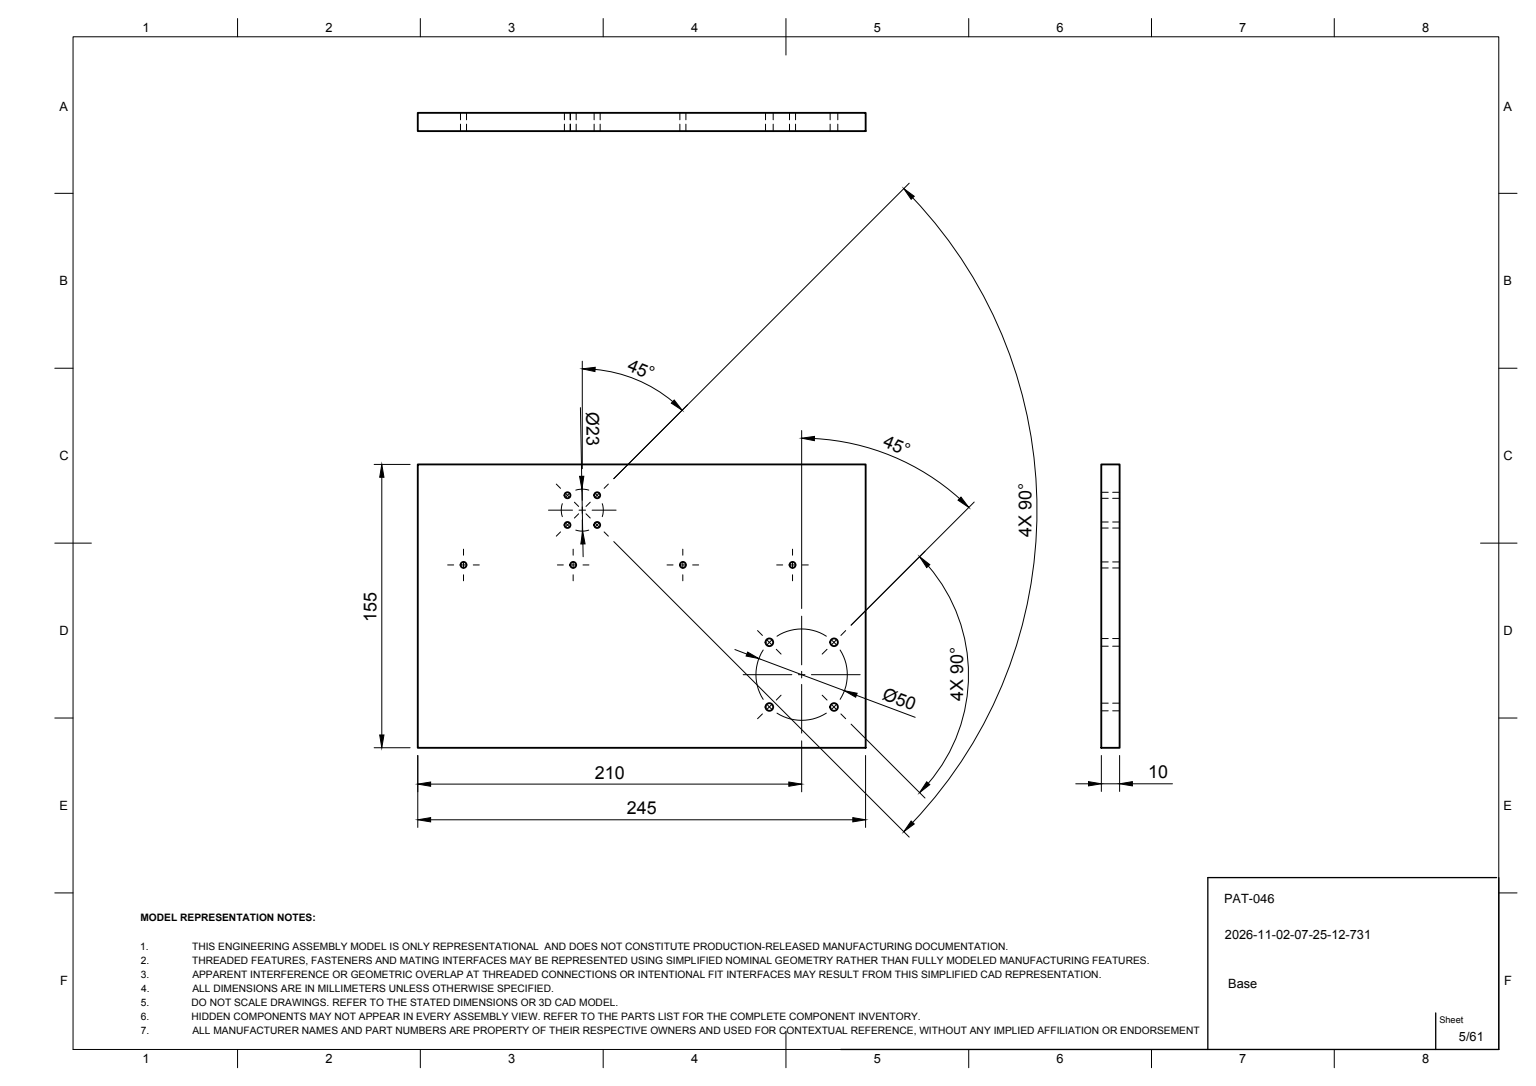
ISO-10303-21;
HEADER;
/* Generated by software containing ST-Developer
 * from STEP Tools, Inc. (www.steptools.com) 
 */

FILE_DESCRIPTION(
/* description */ ('Gear mesh backlash fixture'),
/* implementation_level */ '2;1');

FILE_NAME(
/* name */ 'Base.step',
/* time_stamp */ '2026-10-28T03:26:00-07:00',
/* author */ (''),
/* organization */ (''),
/* preprocessor_version */ 'ST-DEVELOPER v20.2',
/* originating_system */ 'Autodesk Translation Framework v15.17.0.0',
/* authorisation */ '');

FILE_SCHEMA (('AUTOMOTIVE_DESIGN { 1 0 10303 214 3 1 1 }'));
ENDSEC;

DATA;
#10=MECHANICAL_DESIGN_GEOMETRIC_PRESENTATION_REPRESENTATION('',(#1016),#57900);
#916=SHAPE_REPRESENTATION_RELATIONSHIP('SRR','None',#58111,#966);
#966=ADVANCED_BREP_SHAPE_REPRESENTATION('',(#1081),#57844);
#1016=STYLED_ITEM('',(#58444),#1081);
#1081=MANIFOLD_SOLID_BREP('Body1',#13576);
#1143=FACE_BOUND('',#2476,.T.);
#1144=FACE_BOUND('',#2477,.T.);
#1145=FACE_BOUND('',#2478,.T.);
#1146=FACE_BOUND('',#2479,.T.);
#1147=FACE_BOUND('',#2480,.T.);
#1148=FACE_BOUND('',#2481,.T.);
#1149=FACE_BOUND('',#2482,.T.);
#1150=FACE_BOUND('',#2483,.T.);
#1151=FACE_BOUND('',#2484,.T.);
#1152=FACE_BOUND('',#2485,.T.);
#1153=FACE_BOUND('',#2486,.T.);
#1154=FACE_BOUND('',#2487,.T.);
#1155=FACE_BOUND('',#2489,.T.);
#1156=FACE_BOUND('',#2490,.T.);
#1157=FACE_BOUND('',#2491,.T.);
#1158=FACE_BOUND('',#2492,.T.);
#1159=FACE_BOUND('',#2493,.T.);
#1160=FACE_BOUND('',#2494,.T.);
#1161=FACE_BOUND('',#2495,.T.);
#1162=FACE_BOUND('',#2496,.T.);
#1163=FACE_BOUND('',#2497,.T.);
#1164=FACE_BOUND('',#2498,.T.);
#1165=FACE_BOUND('',#2499,.T.);
#1166=FACE_BOUND('',#2500,.T.);
#1330=PLANE('',#14234);
#1331=PLANE('',#14235);
#1332=PLANE('',#14236);
#1333=PLANE('',#14237);
#1334=PLANE('',#14238);
#1335=PLANE('',#14239);
#1694=FACE_OUTER_BOUND('',#2459,.T.);
#1695=FACE_OUTER_BOUND('',#2460,.T.);
#1696=FACE_OUTER_BOUND('',#2461,.T.);
#1697=FACE_OUTER_BOUND('',#2462,.T.);
#1698=FACE_OUTER_BOUND('',#2463,.T.);
#1699=FACE_OUTER_BOUND('',#2464,.T.);
#1700=FACE_OUTER_BOUND('',#2465,.T.);
#1701=FACE_OUTER_BOUND('',#2466,.T.);
#1702=FACE_OUTER_BOUND('',#2467,.T.);
#1703=FACE_OUTER_BOUND('',#2468,.T.);
#1704=FACE_OUTER_BOUND('',#2469,.T.);
#1705=FACE_OUTER_BOUND('',#2470,.T.);
#1706=FACE_OUTER_BOUND('',#2471,.T.);
#1707=FACE_OUTER_BOUND('',#2472,.T.);
#1708=FACE_OUTER_BOUND('',#2473,.T.);
#1709=FACE_OUTER_BOUND('',#2474,.T.);
#1710=FACE_OUTER_BOUND('',#2475,.T.);
#1711=FACE_OUTER_BOUND('',#2488,.T.);
#2459=EDGE_LOOP('',(#8879,#8880,#8881,#8882));
#2460=EDGE_LOOP('',(#8883,#8884,#8885,#8886));
#2461=EDGE_LOOP('',(#8887,#8888,#8889,#8890));
#2462=EDGE_LOOP('',(#8891,#8892,#8893,#8894));
#2463=EDGE_LOOP('',(#8895,#8896,#8897,#8898));
#2464=EDGE_LOOP('',(#8899,#8900,#8901,#8902));
#2465=EDGE_LOOP('',(#8903,#8904,#8905,#8906));
#2466=EDGE_LOOP('',(#8907,#8908,#8909,#8910));
#2467=EDGE_LOOP('',(#8911,#8912,#8913,#8914));
#2468=EDGE_LOOP('',(#8915,#8916,#8917,#8918));
#2469=EDGE_LOOP('',(#8919,#8920,#8921,#8922));
#2470=EDGE_LOOP('',(#8923,#8924,#8925,#8926));
#2471=EDGE_LOOP('',(#8927,#8928,#8929,#8930));
#2472=EDGE_LOOP('',(#8931,#8932,#8933,#8934));
#2473=EDGE_LOOP('',(#8935,#8936,#8937,#8938));
#2474=EDGE_LOOP('',(#8939,#8940,#8941,#8942));
#2475=EDGE_LOOP('',(#8943,#8944,#8945,#8946));
#2476=EDGE_LOOP('',(#8947));
#2477=EDGE_LOOP('',(#8948));
#2478=EDGE_LOOP('',(#8949));
#2479=EDGE_LOOP('',(#8950));
#2480=EDGE_LOOP('',(#8951));
#2481=EDGE_LOOP('',(#8952));
#2482=EDGE_LOOP('',(#8953));
#2483=EDGE_LOOP('',(#8954));
#2484=EDGE_LOOP('',(#8955));
#2485=EDGE_LOOP('',(#8956));
#2486=EDGE_LOOP('',(#8957));
#2487=EDGE_LOOP('',(#8958));
#2488=EDGE_LOOP('',(#8959,#8960,#8961,#8962));
#2489=EDGE_LOOP('',(#8963));
#2490=EDGE_LOOP('',(#8964));
#2491=EDGE_LOOP('',(#8965));
#2492=EDGE_LOOP('',(#8966));
#2493=EDGE_LOOP('',(#8967));
#2494=EDGE_LOOP('',(#8968));
#2495=EDGE_LOOP('',(#8969));
#2496=EDGE_LOOP('',(#8970));
#2497=EDGE_LOOP('',(#8971));
#2498=EDGE_LOOP('',(#8972));
#2499=EDGE_LOOP('',(#8973));
#2500=EDGE_LOOP('',(#8974));
#3411=LINE('',#19240,#4300);
#3412=LINE('',#19246,#4301);
#3413=LINE('',#19252,#4302);
#3414=LINE('',#19258,#4303);
#3415=LINE('',#19264,#4304);
#3416=LINE('',#19270,#4305);
#3417=LINE('',#19276,#4306);
#3418=LINE('',#19282,#4307);
#3419=LINE('',#19288,#4308);
#3420=LINE('',#19294,#4309);
#3421=LINE('',#19300,#4310);
#3422=LINE('',#19306,#4311);
#3423=LINE('',#19311,#4312);
#3424=LINE('',#19313,#4313);
#3425=LINE('',#19315,#4314);
#3426=LINE('',#19316,#4315);
#3427=LINE('',#19319,#4316);
#3428=LINE('',#19321,#4317);
#3429=LINE('',#19322,#4318);
#3430=LINE('',#19325,#4319);
#3431=LINE('',#19327,#4320);
#3432=LINE('',#19328,#4321);
#3433=LINE('',#19330,#4322);
#3434=LINE('',#19331,#4323);
#4300=VECTOR('',#15588,0.164999999999999);
#4301=VECTOR('',#15595,0.164999999999999);
#4302=VECTOR('',#15602,0.164999999999999);
#4303=VECTOR('',#15609,0.164999999999999);
#4304=VECTOR('',#15616,0.21);
#4305=VECTOR('',#15623,0.21);
#4306=VECTOR('',#15630,0.21);
#4307=VECTOR('',#15637,0.21);
#4308=VECTOR('',#15644,0.164999999999999);
#4309=VECTOR('',#15651,0.164999999999999);
#4310=VECTOR('',#15658,0.165);
#4311=VECTOR('',#15665,0.165);
#4312=VECTOR('',#15670,1.);
#4313=VECTOR('',#15671,1.);
#4314=VECTOR('',#15672,1.);
#4315=VECTOR('',#15673,1.);
#4316=VECTOR('',#15676,1.);
#4317=VECTOR('',#15677,1.);
#4318=VECTOR('',#15678,1.);
#4319=VECTOR('',#15681,1.);
#4320=VECTOR('',#15682,1.);
#4321=VECTOR('',#15683,1.);
#4322=VECTOR('',#15686,1.);
#4323=VECTOR('',#15687,1.);
#5189=CIRCLE('',#14199,0.164999999999999);
#5190=CIRCLE('',#14200,0.164999999999999);
#5191=CIRCLE('',#14202,0.164999999999999);
#5192=CIRCLE('',#14203,0.164999999999999);
#5193=CIRCLE('',#14205,0.164999999999999);
#5194=CIRCLE('',#14206,0.164999999999999);
#5195=CIRCLE('',#14208,0.164999999999999);
#5196=CIRCLE('',#14209,0.164999999999999);
#5197=CIRCLE('',#14211,0.21);
#5198=CIRCLE('',#14212,0.21);
#5199=CIRCLE('',#14214,0.21);
#5200=CIRCLE('',#14215,0.21);
#5201=CIRCLE('',#14217,0.21);
#5202=CIRCLE('',#14218,0.21);
#5203=CIRCLE('',#14220,0.21);
#5204=CIRCLE('',#14221,0.21);
#5205=CIRCLE('',#14223,0.164999999999999);
#5206=CIRCLE('',#14224,0.164999999999999);
#5207=CIRCLE('',#14226,0.164999999999999);
#5208=CIRCLE('',#14227,0.164999999999999);
#5209=CIRCLE('',#14229,0.165);
#5210=CIRCLE('',#14230,0.165);
#5211=CIRCLE('',#14232,0.165);
#5212=CIRCLE('',#14233,0.165);
#5781=VERTEX_POINT('',#19237);
#5782=VERTEX_POINT('',#19239);
#5783=VERTEX_POINT('',#19243);
#5784=VERTEX_POINT('',#19245);
#5785=VERTEX_POINT('',#19249);
#5786=VERTEX_POINT('',#19251);
#5787=VERTEX_POINT('',#19255);
#5788=VERTEX_POINT('',#19257);
#5789=VERTEX_POINT('',#19261);
#5790=VERTEX_POINT('',#19263);
#5791=VERTEX_POINT('',#19267);
#5792=VERTEX_POINT('',#19269);
#5793=VERTEX_POINT('',#19273);
#5794=VERTEX_POINT('',#19275);
#5795=VERTEX_POINT('',#19279);
#5796=VERTEX_POINT('',#19281);
#5797=VERTEX_POINT('',#19285);
#5798=VERTEX_POINT('',#19287);
#5799=VERTEX_POINT('',#19291);
#5800=VERTEX_POINT('',#19293);
#5801=VERTEX_POINT('',#19297);
#5802=VERTEX_POINT('',#19299);
#5803=VERTEX_POINT('',#19303);
#5804=VERTEX_POINT('',#19305);
#5805=VERTEX_POINT('',#19309);
#5806=VERTEX_POINT('',#19310);
#5807=VERTEX_POINT('',#19312);
#5808=VERTEX_POINT('',#19314);
#5809=VERTEX_POINT('',#19318);
#5810=VERTEX_POINT('',#19320);
#5811=VERTEX_POINT('',#19324);
#5812=VERTEX_POINT('',#19326);
#7026=EDGE_CURVE('',#5781,#5781,#5189,.T.);
#7027=EDGE_CURVE('',#5781,#5782,#3411,.T.);
#7028=EDGE_CURVE('',#5782,#5782,#5190,.T.);
#7029=EDGE_CURVE('',#5783,#5783,#5191,.T.);
#7030=EDGE_CURVE('',#5783,#5784,#3412,.T.);
#7031=EDGE_CURVE('',#5784,#5784,#5192,.T.);
#7032=EDGE_CURVE('',#5785,#5785,#5193,.T.);
#7033=EDGE_CURVE('',#5785,#5786,#3413,.T.);
#7034=EDGE_CURVE('',#5786,#5786,#5194,.T.);
#7035=EDGE_CURVE('',#5787,#5787,#5195,.T.);
#7036=EDGE_CURVE('',#5787,#5788,#3414,.T.);
#7037=EDGE_CURVE('',#5788,#5788,#5196,.T.);
#7038=EDGE_CURVE('',#5789,#5789,#5197,.T.);
#7039=EDGE_CURVE('',#5789,#5790,#3415,.T.);
#7040=EDGE_CURVE('',#5790,#5790,#5198,.T.);
#7041=EDGE_CURVE('',#5791,#5791,#5199,.T.);
#7042=EDGE_CURVE('',#5791,#5792,#3416,.T.);
#7043=EDGE_CURVE('',#5792,#5792,#5200,.T.);
#7044=EDGE_CURVE('',#5793,#5793,#5201,.T.);
#7045=EDGE_CURVE('',#5793,#5794,#3417,.T.);
#7046=EDGE_CURVE('',#5794,#5794,#5202,.T.);
#7047=EDGE_CURVE('',#5795,#5795,#5203,.T.);
#7048=EDGE_CURVE('',#5795,#5796,#3418,.T.);
#7049=EDGE_CURVE('',#5796,#5796,#5204,.T.);
#7050=EDGE_CURVE('',#5797,#5797,#5205,.T.);
#7051=EDGE_CURVE('',#5797,#5798,#3419,.T.);
#7052=EDGE_CURVE('',#5798,#5798,#5206,.T.);
#7053=EDGE_CURVE('',#5799,#5799,#5207,.T.);
#7054=EDGE_CURVE('',#5799,#5800,#3420,.T.);
#7055=EDGE_CURVE('',#5800,#5800,#5208,.T.);
#7056=EDGE_CURVE('',#5801,#5801,#5209,.T.);
#7057=EDGE_CURVE('',#5801,#5802,#3421,.T.);
#7058=EDGE_CURVE('',#5802,#5802,#5210,.T.);
#7059=EDGE_CURVE('',#5803,#5803,#5211,.T.);
#7060=EDGE_CURVE('',#5803,#5804,#3422,.T.);
#7061=EDGE_CURVE('',#5804,#5804,#5212,.T.);
#7062=EDGE_CURVE('',#5805,#5806,#3423,.T.);
#7063=EDGE_CURVE('',#5806,#5807,#3424,.T.);
#7064=EDGE_CURVE('',#5808,#5807,#3425,.T.);
#7065=EDGE_CURVE('',#5805,#5808,#3426,.T.);
#7066=EDGE_CURVE('',#5809,#5805,#3427,.T.);
#7067=EDGE_CURVE('',#5810,#5808,#3428,.T.);
#7068=EDGE_CURVE('',#5809,#5810,#3429,.T.);
#7069=EDGE_CURVE('',#5811,#5809,#3430,.T.);
#7070=EDGE_CURVE('',#5812,#5810,#3431,.T.);
#7071=EDGE_CURVE('',#5811,#5812,#3432,.T.);
#7072=EDGE_CURVE('',#5806,#5811,#3433,.T.);
#7073=EDGE_CURVE('',#5807,#5812,#3434,.T.);
#8879=ORIENTED_EDGE('',*,*,#7026,.F.);
#8880=ORIENTED_EDGE('',*,*,#7027,.T.);
#8881=ORIENTED_EDGE('',*,*,#7028,.F.);
#8882=ORIENTED_EDGE('',*,*,#7027,.F.);
#8883=ORIENTED_EDGE('',*,*,#7029,.F.);
#8884=ORIENTED_EDGE('',*,*,#7030,.T.);
#8885=ORIENTED_EDGE('',*,*,#7031,.F.);
#8886=ORIENTED_EDGE('',*,*,#7030,.F.);
#8887=ORIENTED_EDGE('',*,*,#7032,.F.);
#8888=ORIENTED_EDGE('',*,*,#7033,.T.);
#8889=ORIENTED_EDGE('',*,*,#7034,.F.);
#8890=ORIENTED_EDGE('',*,*,#7033,.F.);
#8891=ORIENTED_EDGE('',*,*,#7035,.F.);
#8892=ORIENTED_EDGE('',*,*,#7036,.T.);
#8893=ORIENTED_EDGE('',*,*,#7037,.F.);
#8894=ORIENTED_EDGE('',*,*,#7036,.F.);
#8895=ORIENTED_EDGE('',*,*,#7038,.F.);
#8896=ORIENTED_EDGE('',*,*,#7039,.T.);
#8897=ORIENTED_EDGE('',*,*,#7040,.F.);
#8898=ORIENTED_EDGE('',*,*,#7039,.F.);
#8899=ORIENTED_EDGE('',*,*,#7041,.F.);
#8900=ORIENTED_EDGE('',*,*,#7042,.T.);
#8901=ORIENTED_EDGE('',*,*,#7043,.F.);
#8902=ORIENTED_EDGE('',*,*,#7042,.F.);
#8903=ORIENTED_EDGE('',*,*,#7044,.F.);
#8904=ORIENTED_EDGE('',*,*,#7045,.T.);
#8905=ORIENTED_EDGE('',*,*,#7046,.F.);
#8906=ORIENTED_EDGE('',*,*,#7045,.F.);
#8907=ORIENTED_EDGE('',*,*,#7047,.F.);
#8908=ORIENTED_EDGE('',*,*,#7048,.T.);
#8909=ORIENTED_EDGE('',*,*,#7049,.F.);
#8910=ORIENTED_EDGE('',*,*,#7048,.F.);
#8911=ORIENTED_EDGE('',*,*,#7050,.F.);
#8912=ORIENTED_EDGE('',*,*,#7051,.T.);
#8913=ORIENTED_EDGE('',*,*,#7052,.F.);
#8914=ORIENTED_EDGE('',*,*,#7051,.F.);
#8915=ORIENTED_EDGE('',*,*,#7053,.F.);
#8916=ORIENTED_EDGE('',*,*,#7054,.T.);
#8917=ORIENTED_EDGE('',*,*,#7055,.F.);
#8918=ORIENTED_EDGE('',*,*,#7054,.F.);
#8919=ORIENTED_EDGE('',*,*,#7056,.F.);
#8920=ORIENTED_EDGE('',*,*,#7057,.T.);
#8921=ORIENTED_EDGE('',*,*,#7058,.F.);
#8922=ORIENTED_EDGE('',*,*,#7057,.F.);
#8923=ORIENTED_EDGE('',*,*,#7059,.F.);
#8924=ORIENTED_EDGE('',*,*,#7060,.T.);
#8925=ORIENTED_EDGE('',*,*,#7061,.F.);
#8926=ORIENTED_EDGE('',*,*,#7060,.F.);
#8927=ORIENTED_EDGE('',*,*,#7062,.T.);
#8928=ORIENTED_EDGE('',*,*,#7063,.T.);
#8929=ORIENTED_EDGE('',*,*,#7064,.F.);
#8930=ORIENTED_EDGE('',*,*,#7065,.F.);
#8931=ORIENTED_EDGE('',*,*,#7066,.T.);
#8932=ORIENTED_EDGE('',*,*,#7065,.T.);
#8933=ORIENTED_EDGE('',*,*,#7067,.F.);
#8934=ORIENTED_EDGE('',*,*,#7068,.F.);
#8935=ORIENTED_EDGE('',*,*,#7069,.T.);
#8936=ORIENTED_EDGE('',*,*,#7068,.T.);
#8937=ORIENTED_EDGE('',*,*,#7070,.F.);
#8938=ORIENTED_EDGE('',*,*,#7071,.F.);
#8939=ORIENTED_EDGE('',*,*,#7072,.T.);
#8940=ORIENTED_EDGE('',*,*,#7071,.T.);
#8941=ORIENTED_EDGE('',*,*,#7073,.F.);
#8942=ORIENTED_EDGE('',*,*,#7063,.F.);
#8943=ORIENTED_EDGE('',*,*,#7073,.T.);
#8944=ORIENTED_EDGE('',*,*,#7070,.T.);
#8945=ORIENTED_EDGE('',*,*,#7067,.T.);
#8946=ORIENTED_EDGE('',*,*,#7064,.T.);
#8947=ORIENTED_EDGE('',*,*,#7040,.T.);
#8948=ORIENTED_EDGE('',*,*,#7043,.T.);
#8949=ORIENTED_EDGE('',*,*,#7046,.T.);
#8950=ORIENTED_EDGE('',*,*,#7049,.T.);
#8951=ORIENTED_EDGE('',*,*,#7052,.T.);
#8952=ORIENTED_EDGE('',*,*,#7055,.T.);
#8953=ORIENTED_EDGE('',*,*,#7058,.T.);
#8954=ORIENTED_EDGE('',*,*,#7061,.T.);
#8955=ORIENTED_EDGE('',*,*,#7037,.T.);
#8956=ORIENTED_EDGE('',*,*,#7034,.T.);
#8957=ORIENTED_EDGE('',*,*,#7031,.T.);
#8958=ORIENTED_EDGE('',*,*,#7028,.T.);
#8959=ORIENTED_EDGE('',*,*,#7072,.F.);
#8960=ORIENTED_EDGE('',*,*,#7062,.F.);
#8961=ORIENTED_EDGE('',*,*,#7066,.F.);
#8962=ORIENTED_EDGE('',*,*,#7069,.F.);
#8963=ORIENTED_EDGE('',*,*,#7038,.T.);
#8964=ORIENTED_EDGE('',*,*,#7041,.T.);
#8965=ORIENTED_EDGE('',*,*,#7044,.T.);
#8966=ORIENTED_EDGE('',*,*,#7047,.T.);
#8967=ORIENTED_EDGE('',*,*,#7050,.T.);
#8968=ORIENTED_EDGE('',*,*,#7053,.T.);
#8969=ORIENTED_EDGE('',*,*,#7056,.T.);
#8970=ORIENTED_EDGE('',*,*,#7059,.T.);
#8971=ORIENTED_EDGE('',*,*,#7035,.T.);
#8972=ORIENTED_EDGE('',*,*,#7032,.T.);
#8973=ORIENTED_EDGE('',*,*,#7029,.T.);
#8974=ORIENTED_EDGE('',*,*,#7026,.T.);
#12585=CYLINDRICAL_SURFACE('',#14198,0.164999999999999);
#12586=CYLINDRICAL_SURFACE('',#14201,0.164999999999999);
#12587=CYLINDRICAL_SURFACE('',#14204,0.164999999999999);
#12588=CYLINDRICAL_SURFACE('',#14207,0.164999999999999);
#12589=CYLINDRICAL_SURFACE('',#14210,0.21);
#12590=CYLINDRICAL_SURFACE('',#14213,0.21);
#12591=CYLINDRICAL_SURFACE('',#14216,0.21);
#12592=CYLINDRICAL_SURFACE('',#14219,0.21);
#12593=CYLINDRICAL_SURFACE('',#14222,0.164999999999999);
#12594=CYLINDRICAL_SURFACE('',#14225,0.164999999999999);
#12595=CYLINDRICAL_SURFACE('',#14228,0.165);
#12596=CYLINDRICAL_SURFACE('',#14231,0.165);
#12811=ADVANCED_FACE('',(#1694),#12585,.F.);
#12812=ADVANCED_FACE('',(#1695),#12586,.F.);
#12813=ADVANCED_FACE('',(#1696),#12587,.F.);
#12814=ADVANCED_FACE('',(#1697),#12588,.F.);
#12815=ADVANCED_FACE('',(#1698),#12589,.F.);
#12816=ADVANCED_FACE('',(#1699),#12590,.F.);
#12817=ADVANCED_FACE('',(#1700),#12591,.F.);
#12818=ADVANCED_FACE('',(#1701),#12592,.F.);
#12819=ADVANCED_FACE('',(#1702),#12593,.F.);
#12820=ADVANCED_FACE('',(#1703),#12594,.F.);
#12821=ADVANCED_FACE('',(#1704),#12595,.F.);
#12822=ADVANCED_FACE('',(#1705),#12596,.F.);
#12823=ADVANCED_FACE('',(#1706),#1330,.T.);
#12824=ADVANCED_FACE('',(#1707),#1331,.T.);
#12825=ADVANCED_FACE('',(#1708),#1332,.T.);
#12826=ADVANCED_FACE('',(#1709),#1333,.T.);
#12827=ADVANCED_FACE('',(#1710,#1143,#1144,#1145,#1146,#1147,#1148,#1149,
#1150,#1151,#1152,#1153,#1154),#1334,.T.);
#12828=ADVANCED_FACE('',(#1711,#1155,#1156,#1157,#1158,#1159,#1160,#1161,
#1162,#1163,#1164,#1165,#1166),#1335,.F.);
#13576=CLOSED_SHELL('',(#12811,#12812,#12813,#12814,#12815,#12816,#12817,
#12818,#12819,#12820,#12821,#12822,#12823,#12824,#12825,#12826,#12827,#12828));
#14197=AXIS2_PLACEMENT_3D('',#19235,#15582,#15583);
#14198=AXIS2_PLACEMENT_3D('',#19236,#15584,#15585);
#14199=AXIS2_PLACEMENT_3D('',#19238,#15586,#15587);
#14200=AXIS2_PLACEMENT_3D('',#19241,#15589,#15590);
#14201=AXIS2_PLACEMENT_3D('',#19242,#15591,#15592);
#14202=AXIS2_PLACEMENT_3D('',#19244,#15593,#15594);
#14203=AXIS2_PLACEMENT_3D('',#19247,#15596,#15597);
#14204=AXIS2_PLACEMENT_3D('',#19248,#15598,#15599);
#14205=AXIS2_PLACEMENT_3D('',#19250,#15600,#15601);
#14206=AXIS2_PLACEMENT_3D('',#19253,#15603,#15604);
#14207=AXIS2_PLACEMENT_3D('',#19254,#15605,#15606);
#14208=AXIS2_PLACEMENT_3D('',#19256,#15607,#15608);
#14209=AXIS2_PLACEMENT_3D('',#19259,#15610,#15611);
#14210=AXIS2_PLACEMENT_3D('',#19260,#15612,#15613);
#14211=AXIS2_PLACEMENT_3D('',#19262,#15614,#15615);
#14212=AXIS2_PLACEMENT_3D('',#19265,#15617,#15618);
#14213=AXIS2_PLACEMENT_3D('',#19266,#15619,#15620);
#14214=AXIS2_PLACEMENT_3D('',#19268,#15621,#15622);
#14215=AXIS2_PLACEMENT_3D('',#19271,#15624,#15625);
#14216=AXIS2_PLACEMENT_3D('',#19272,#15626,#15627);
#14217=AXIS2_PLACEMENT_3D('',#19274,#15628,#15629);
#14218=AXIS2_PLACEMENT_3D('',#19277,#15631,#15632);
#14219=AXIS2_PLACEMENT_3D('',#19278,#15633,#15634);
#14220=AXIS2_PLACEMENT_3D('',#19280,#15635,#15636);
#14221=AXIS2_PLACEMENT_3D('',#19283,#15638,#15639);
#14222=AXIS2_PLACEMENT_3D('',#19284,#15640,#15641);
#14223=AXIS2_PLACEMENT_3D('',#19286,#15642,#15643);
#14224=AXIS2_PLACEMENT_3D('',#19289,#15645,#15646);
#14225=AXIS2_PLACEMENT_3D('',#19290,#15647,#15648);
#14226=AXIS2_PLACEMENT_3D('',#19292,#15649,#15650);
#14227=AXIS2_PLACEMENT_3D('',#19295,#15652,#15653);
#14228=AXIS2_PLACEMENT_3D('',#19296,#15654,#15655);
#14229=AXIS2_PLACEMENT_3D('',#19298,#15656,#15657);
#14230=AXIS2_PLACEMENT_3D('',#19301,#15659,#15660);
#14231=AXIS2_PLACEMENT_3D('',#19302,#15661,#15662);
#14232=AXIS2_PLACEMENT_3D('',#19304,#15663,#15664);
#14233=AXIS2_PLACEMENT_3D('',#19307,#15666,#15667);
#14234=AXIS2_PLACEMENT_3D('',#19308,#15668,#15669);
#14235=AXIS2_PLACEMENT_3D('',#19317,#15674,#15675);
#14236=AXIS2_PLACEMENT_3D('',#19323,#15679,#15680);
#14237=AXIS2_PLACEMENT_3D('',#19329,#15684,#15685);
#14238=AXIS2_PLACEMENT_3D('',#19332,#15688,#15689);
#14239=AXIS2_PLACEMENT_3D('',#19333,#15690,#15691);
#15582=DIRECTION('axis',(0.,0.,1.));
#15583=DIRECTION('refdir',(1.,0.,0.));
#15584=DIRECTION('center_axis',(0.,0.,1.));
#15585=DIRECTION('ref_axis',(1.,0.,0.));
#15586=DIRECTION('center_axis',(0.,0.,1.));
#15587=DIRECTION('ref_axis',(1.,0.,0.));
#15588=DIRECTION('',(0.,0.,1.));
#15589=DIRECTION('center_axis',(0.,0.,-1.));
#15590=DIRECTION('ref_axis',(1.,0.,0.));
#15591=DIRECTION('center_axis',(0.,0.,1.));
#15592=DIRECTION('ref_axis',(1.,0.,0.));
#15593=DIRECTION('center_axis',(0.,0.,1.));
#15594=DIRECTION('ref_axis',(1.,0.,0.));
#15595=DIRECTION('',(0.,0.,1.));
#15596=DIRECTION('center_axis',(0.,0.,-1.));
#15597=DIRECTION('ref_axis',(1.,0.,0.));
#15598=DIRECTION('center_axis',(0.,0.,1.));
#15599=DIRECTION('ref_axis',(1.,0.,0.));
#15600=DIRECTION('center_axis',(0.,0.,1.));
#15601=DIRECTION('ref_axis',(1.,0.,0.));
#15602=DIRECTION('',(0.,0.,1.));
#15603=DIRECTION('center_axis',(0.,0.,-1.));
#15604=DIRECTION('ref_axis',(1.,0.,0.));
#15605=DIRECTION('center_axis',(0.,0.,1.));
#15606=DIRECTION('ref_axis',(1.,0.,0.));
#15607=DIRECTION('center_axis',(0.,0.,1.));
#15608=DIRECTION('ref_axis',(1.,0.,0.));
#15609=DIRECTION('',(0.,0.,1.));
#15610=DIRECTION('center_axis',(0.,0.,-1.));
#15611=DIRECTION('ref_axis',(1.,0.,0.));
#15612=DIRECTION('center_axis',(0.,0.,1.));
#15613=DIRECTION('ref_axis',(1.,0.,0.));
#15614=DIRECTION('center_axis',(0.,0.,1.));
#15615=DIRECTION('ref_axis',(1.,0.,0.));
#15616=DIRECTION('',(0.,0.,1.));
#15617=DIRECTION('center_axis',(0.,0.,-1.));
#15618=DIRECTION('ref_axis',(1.,0.,0.));
#15619=DIRECTION('center_axis',(0.,0.,1.));
#15620=DIRECTION('ref_axis',(1.,0.,0.));
#15621=DIRECTION('center_axis',(0.,0.,1.));
#15622=DIRECTION('ref_axis',(1.,0.,0.));
#15623=DIRECTION('',(0.,0.,1.));
#15624=DIRECTION('center_axis',(0.,0.,-1.));
#15625=DIRECTION('ref_axis',(1.,0.,0.));
#15626=DIRECTION('center_axis',(0.,0.,1.));
#15627=DIRECTION('ref_axis',(1.,0.,0.));
#15628=DIRECTION('center_axis',(0.,0.,1.));
#15629=DIRECTION('ref_axis',(1.,0.,0.));
#15630=DIRECTION('',(0.,0.,1.));
#15631=DIRECTION('center_axis',(0.,0.,-1.));
#15632=DIRECTION('ref_axis',(1.,0.,0.));
#15633=DIRECTION('center_axis',(0.,0.,1.));
#15634=DIRECTION('ref_axis',(1.,0.,0.));
#15635=DIRECTION('center_axis',(0.,0.,1.));
#15636=DIRECTION('ref_axis',(1.,0.,0.));
#15637=DIRECTION('',(0.,0.,1.));
#15638=DIRECTION('center_axis',(0.,0.,-1.));
#15639=DIRECTION('ref_axis',(1.,0.,0.));
#15640=DIRECTION('center_axis',(0.,0.,1.));
#15641=DIRECTION('ref_axis',(1.,0.,0.));
#15642=DIRECTION('center_axis',(0.,0.,1.));
#15643=DIRECTION('ref_axis',(1.,0.,0.));
#15644=DIRECTION('',(0.,0.,1.));
#15645=DIRECTION('center_axis',(0.,0.,-1.));
#15646=DIRECTION('ref_axis',(1.,0.,0.));
#15647=DIRECTION('center_axis',(0.,0.,1.));
#15648=DIRECTION('ref_axis',(1.,0.,0.));
#15649=DIRECTION('center_axis',(0.,0.,1.));
#15650=DIRECTION('ref_axis',(1.,0.,0.));
#15651=DIRECTION('',(0.,0.,1.));
#15652=DIRECTION('center_axis',(0.,0.,-1.));
#15653=DIRECTION('ref_axis',(1.,0.,0.));
#15654=DIRECTION('center_axis',(0.,0.,1.));
#15655=DIRECTION('ref_axis',(1.,0.,0.));
#15656=DIRECTION('center_axis',(0.,0.,1.));
#15657=DIRECTION('ref_axis',(1.,0.,0.));
#15658=DIRECTION('',(0.,0.,1.));
#15659=DIRECTION('center_axis',(0.,0.,-1.));
#15660=DIRECTION('ref_axis',(1.,0.,0.));
#15661=DIRECTION('center_axis',(0.,0.,1.));
#15662=DIRECTION('ref_axis',(1.,0.,0.));
#15663=DIRECTION('center_axis',(0.,0.,1.));
#15664=DIRECTION('ref_axis',(1.,0.,0.));
#15665=DIRECTION('',(0.,0.,1.));
#15666=DIRECTION('center_axis',(0.,0.,-1.));
#15667=DIRECTION('ref_axis',(1.,0.,0.));
#15668=DIRECTION('center_axis',(0.,1.,0.));
#15669=DIRECTION('ref_axis',(-1.,0.,0.));
#15670=DIRECTION('',(-1.,0.,0.));
#15671=DIRECTION('',(0.,0.,1.));
#15672=DIRECTION('',(-1.,0.,0.));
#15673=DIRECTION('',(0.,0.,1.));
#15674=DIRECTION('center_axis',(1.,0.,0.));
#15675=DIRECTION('ref_axis',(0.,1.,0.));
#15676=DIRECTION('',(0.,1.,0.));
#15677=DIRECTION('',(0.,1.,0.));
#15678=DIRECTION('',(0.,0.,1.));
#15679=DIRECTION('center_axis',(0.,-1.,0.));
#15680=DIRECTION('ref_axis',(1.,0.,0.));
#15681=DIRECTION('',(1.,0.,0.));
#15682=DIRECTION('',(1.,0.,0.));
#15683=DIRECTION('',(0.,0.,1.));
#15684=DIRECTION('center_axis',(-1.,0.,0.));
#15685=DIRECTION('ref_axis',(0.,-1.,0.));
#15686=DIRECTION('',(0.,-1.,0.));
#15687=DIRECTION('',(0.,-1.,0.));
#15688=DIRECTION('center_axis',(0.,0.,1.));
#15689=DIRECTION('ref_axis',(1.,0.,0.));
#15690=DIRECTION('center_axis',(0.,0.,1.));
#15691=DIRECTION('ref_axis',(1.,0.,0.));
#19235=CARTESIAN_POINT('',(0.,0.,0.));
#19236=CARTESIAN_POINT('Origin',(11.1868272016355,8.18682720163547,-1.1));
#19237=CARTESIAN_POINT('',(11.0218272016355,8.18682720163547,-1.));
#19238=CARTESIAN_POINT('Origin',(11.1868272016355,8.18682720163547,-1.));
#19239=CARTESIAN_POINT('',(11.0218272016355,8.18682720163547,0.));
#19240=CARTESIAN_POINT('',(11.0218272016355,8.18682720163547,-1.1));
#19241=CARTESIAN_POINT('Origin',(11.1868272016355,8.18682720163547,0.));
#19242=CARTESIAN_POINT('Origin',(11.1868272016355,9.81317279836453,-1.1));
#19243=CARTESIAN_POINT('',(11.0218272016355,9.81317279836453,-1.));
#19244=CARTESIAN_POINT('Origin',(11.1868272016355,9.81317279836453,-1.));
#19245=CARTESIAN_POINT('',(11.0218272016355,9.81317279836453,0.));
#19246=CARTESIAN_POINT('',(11.0218272016355,9.81317279836453,-1.1));
#19247=CARTESIAN_POINT('Origin',(11.1868272016355,9.81317279836453,0.));
#19248=CARTESIAN_POINT('Origin',(12.8131727983645,9.81317279836453,-1.1));
#19249=CARTESIAN_POINT('',(12.6481727983645,9.81317279836453,-1.));
#19250=CARTESIAN_POINT('Origin',(12.8131727983645,9.81317279836453,-1.));
#19251=CARTESIAN_POINT('',(12.6481727983645,9.81317279836453,0.));
#19252=CARTESIAN_POINT('',(12.6481727983645,9.81317279836453,-1.1));
#19253=CARTESIAN_POINT('Origin',(12.8131727983645,9.81317279836453,0.));
#19254=CARTESIAN_POINT('Origin',(12.8131727983645,8.18682720163547,-1.1));
#19255=CARTESIAN_POINT('',(12.6481727983645,8.18682720163547,-1.));
#19256=CARTESIAN_POINT('Origin',(12.8131727983645,8.18682720163547,-1.));
#19257=CARTESIAN_POINT('',(12.6481727983645,8.18682720163547,0.));
#19258=CARTESIAN_POINT('',(12.6481727983645,8.18682720163547,-1.1));
#19259=CARTESIAN_POINT('Origin',(12.8131727983645,8.18682720163547,0.));
#19260=CARTESIAN_POINT('Origin',(-1.76776695296637,-1.76776695296637,-1.1));
#19261=CARTESIAN_POINT('',(-1.97776695296637,-1.76776695296637,-1.));
#19262=CARTESIAN_POINT('Origin',(-1.76776695296637,-1.76776695296637,-1.));
#19263=CARTESIAN_POINT('',(-1.97776695296637,-1.76776695296637,0.));
#19264=CARTESIAN_POINT('',(-1.97776695296637,-1.76776695296637,-1.1));
#19265=CARTESIAN_POINT('Origin',(-1.76776695296637,-1.76776695296637,0.));
#19266=CARTESIAN_POINT('Origin',(-1.76776695296637,1.76776695296637,-1.1));
#19267=CARTESIAN_POINT('',(-1.97776695296637,1.76776695296637,-1.));
#19268=CARTESIAN_POINT('Origin',(-1.76776695296637,1.76776695296637,-1.));
#19269=CARTESIAN_POINT('',(-1.97776695296637,1.76776695296637,0.));
#19270=CARTESIAN_POINT('',(-1.97776695296637,1.76776695296637,-1.1));
#19271=CARTESIAN_POINT('Origin',(-1.76776695296637,1.76776695296637,0.));
#19272=CARTESIAN_POINT('Origin',(1.76776695296637,1.76776695296637,-1.1));
#19273=CARTESIAN_POINT('',(1.55776695296637,1.76776695296637,-1.));
#19274=CARTESIAN_POINT('Origin',(1.76776695296637,1.76776695296637,-1.));
#19275=CARTESIAN_POINT('',(1.55776695296637,1.76776695296637,0.));
#19276=CARTESIAN_POINT('',(1.55776695296637,1.76776695296637,-1.1));
#19277=CARTESIAN_POINT('Origin',(1.76776695296637,1.76776695296637,0.));
#19278=CARTESIAN_POINT('Origin',(1.76776695296637,-1.76776695296637,-1.1));
#19279=CARTESIAN_POINT('',(1.55776695296637,-1.76776695296637,-1.));
#19280=CARTESIAN_POINT('Origin',(1.76776695296637,-1.76776695296637,-1.));
#19281=CARTESIAN_POINT('',(1.55776695296637,-1.76776695296637,0.));
#19282=CARTESIAN_POINT('',(1.55776695296637,-1.76776695296637,-1.1));
#19283=CARTESIAN_POINT('Origin',(1.76776695296637,-1.76776695296637,0.));
#19284=CARTESIAN_POINT('Origin',(18.5,6.,-1.1));
#19285=CARTESIAN_POINT('',(18.335,6.,-1.));
#19286=CARTESIAN_POINT('Origin',(18.5,6.,-1.));
#19287=CARTESIAN_POINT('',(18.335,6.,0.));
#19288=CARTESIAN_POINT('',(18.335,6.,-1.1));
#19289=CARTESIAN_POINT('Origin',(18.5,6.,0.));
#19290=CARTESIAN_POINT('Origin',(12.5,6.,-1.1));
#19291=CARTESIAN_POINT('',(12.335,6.,-1.));
#19292=CARTESIAN_POINT('Origin',(12.5,6.,-1.));
#19293=CARTESIAN_POINT('',(12.335,6.,0.));
#19294=CARTESIAN_POINT('',(12.335,6.,-1.1));
#19295=CARTESIAN_POINT('Origin',(12.5,6.,0.));
#19296=CARTESIAN_POINT('Origin',(6.5,6.,-1.1));
#19297=CARTESIAN_POINT('',(6.335,6.,-1.));
#19298=CARTESIAN_POINT('Origin',(6.5,6.,-1.));
#19299=CARTESIAN_POINT('',(6.335,6.,0.));
#19300=CARTESIAN_POINT('',(6.335,6.,-1.1));
#19301=CARTESIAN_POINT('Origin',(6.5,6.,0.));
#19302=CARTESIAN_POINT('Origin',(0.5,6.,-1.1));
#19303=CARTESIAN_POINT('',(0.335,6.,-1.));
#19304=CARTESIAN_POINT('Origin',(0.5,6.,-1.));
#19305=CARTESIAN_POINT('',(0.335,6.,0.));
#19306=CARTESIAN_POINT('',(0.335,6.,-1.1));
#19307=CARTESIAN_POINT('Origin',(0.5,6.,0.));
#19308=CARTESIAN_POINT('Origin',(21.,11.5,-1.));
#19309=CARTESIAN_POINT('',(21.,11.5,-1.));
#19310=CARTESIAN_POINT('',(-3.5,11.5,-1.));
#19311=CARTESIAN_POINT('',(21.,11.5,-1.));
#19312=CARTESIAN_POINT('',(-3.5,11.5,0.));
#19313=CARTESIAN_POINT('',(-3.5,11.5,-1.));
#19314=CARTESIAN_POINT('',(21.,11.5,0.));
#19315=CARTESIAN_POINT('',(21.,11.5,0.));
#19316=CARTESIAN_POINT('',(21.,11.5,-1.));
#19317=CARTESIAN_POINT('Origin',(21.,-4.,-1.));
#19318=CARTESIAN_POINT('',(21.,-4.,-1.));
#19319=CARTESIAN_POINT('',(21.,-4.,-1.));
#19320=CARTESIAN_POINT('',(21.,-4.,0.));
#19321=CARTESIAN_POINT('',(21.,-4.,0.));
#19322=CARTESIAN_POINT('',(21.,-4.,-1.));
#19323=CARTESIAN_POINT('Origin',(-3.5,-4.,-1.));
#19324=CARTESIAN_POINT('',(-3.5,-4.,-1.));
#19325=CARTESIAN_POINT('',(-3.5,-4.,-1.));
#19326=CARTESIAN_POINT('',(-3.5,-4.,0.));
#19327=CARTESIAN_POINT('',(-3.5,-4.,0.));
#19328=CARTESIAN_POINT('',(-3.5,-4.,-1.));
#19329=CARTESIAN_POINT('Origin',(-3.5,11.5,-1.));
#19330=CARTESIAN_POINT('',(-3.5,11.5,-1.));
#19331=CARTESIAN_POINT('',(-3.5,11.5,0.));
#19332=CARTESIAN_POINT('Origin',(8.75,3.75,0.));
#19333=CARTESIAN_POINT('Origin',(8.75,3.75,-1.));
#57785=UNCERTAINTY_MEASURE_WITH_UNIT(LENGTH_MEASURE(0.001),#57901,
'DISTANCE_ACCURACY_VALUE',
'Maximum model space distance between geometric entities at asserted c
onnectivities');
#57841=UNCERTAINTY_MEASURE_WITH_UNIT(LENGTH_MEASURE(0.001),#57901,
'DISTANCE_ACCURACY_VALUE',
'Maximum model space distance between geometric entities at asserted c
onnectivities');
#57844=(
GEOMETRIC_REPRESENTATION_CONTEXT(3)
GLOBAL_UNCERTAINTY_ASSIGNED_CONTEXT((#57785))
GLOBAL_UNIT_ASSIGNED_CONTEXT((#57901,#57903,#57904))
REPRESENTATION_CONTEXT('','3D')
);
#57900=(
GEOMETRIC_REPRESENTATION_CONTEXT(3)
GLOBAL_UNCERTAINTY_ASSIGNED_CONTEXT((#57841))
GLOBAL_UNIT_ASSIGNED_CONTEXT((#57901,#57903,#57904))
REPRESENTATION_CONTEXT('','3D')
);
#57901=(
LENGTH_UNIT()
NAMED_UNIT(*)
SI_UNIT(.CENTI.,.METRE.)
);
#57903=(
NAMED_UNIT(*)
PLANE_ANGLE_UNIT()
SI_UNIT($,.RADIAN.)
);
#57904=(
NAMED_UNIT(*)
SI_UNIT($,.STERADIAN.)
SOLID_ANGLE_UNIT()
);
#57907=SHAPE_DEFINITION_REPRESENTATION(#57965,#58111);
#57965=PRODUCT_DEFINITION_SHAPE('',$,#58170);
#58111=SHAPE_REPRESENTATION('',(#14197),#57844);
#58167=PRODUCT_DEFINITION_CONTEXT('part definition',#58343,'design');
#58170=PRODUCT_DEFINITION('Base','Base',#58228,#58167);
#58228=PRODUCT_DEFINITION_FORMATION('',$,#58347);
#58343=APPLICATION_CONTEXT(
'Core Data for Automotive Mechanical Design Process');
#58344=PRODUCT_CONTEXT('part definition',#58343,'mechanical');
#58347=PRODUCT('Base','Base','Base',(#58344));
#58438=COLOUR_RGB('Dark Blue',0.08,0.2,0.34);
#58439=FILL_AREA_STYLE_COLOUR('',#58438);
#58440=FILL_AREA_STYLE('',(#58439));
#58441=SURFACE_STYLE_FILL_AREA(#58440);
#58442=SURFACE_SIDE_STYLE('',(#58441));
#58443=SURFACE_STYLE_USAGE(.BOTH.,#58442);
#58444=PRESENTATION_STYLE_ASSIGNMENT((#58443));
ENDSEC;
END-ISO-10303-21;
